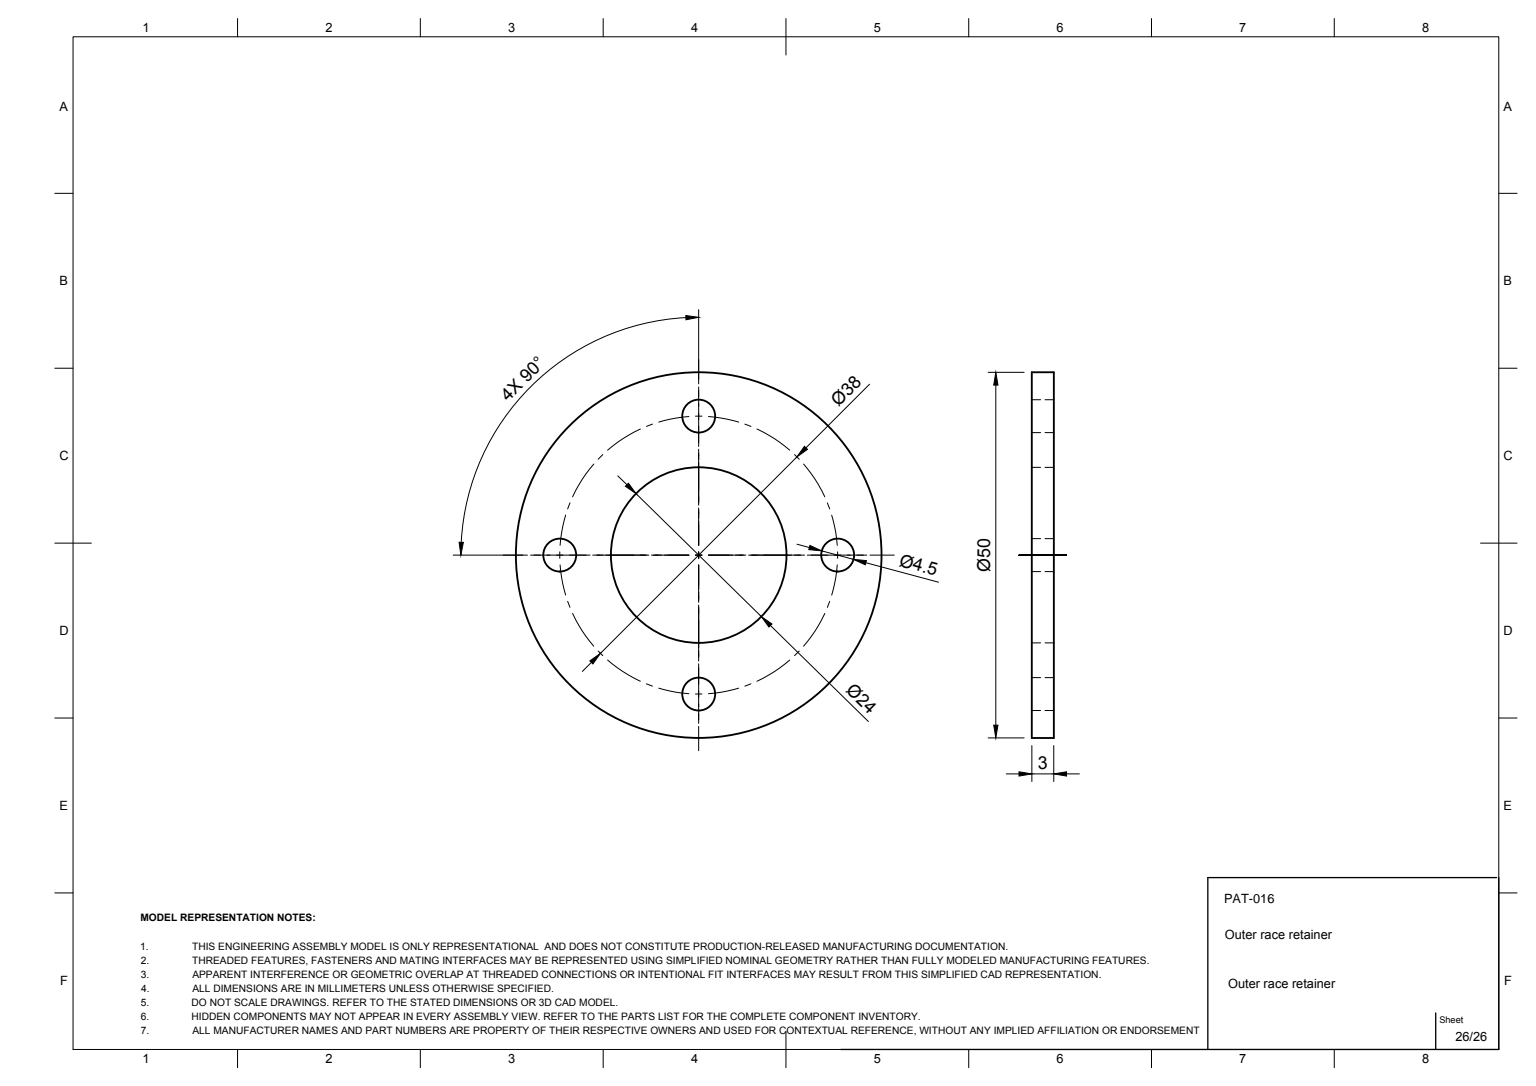
ISO-10303-21;
HEADER;
/* Generated by software containing ST-Developer
 * from STEP Tools, Inc. (www.steptools.com) 
 */

FILE_DESCRIPTION(
/* description */ ('Bracket-mounted idler roller'),
/* implementation_level */ '2;1');

FILE_NAME(
/* name */ 'Outer race retainer.step',
/* time_stamp */ '2026-10-28T03:26:42-07:00',
/* author */ (''),
/* organization */ (''),
/* preprocessor_version */ 'ST-DEVELOPER v20.2',
/* originating_system */ 'Autodesk Translation Framework v15.17.0.0',
/* authorisation */ '');

FILE_SCHEMA (('AUTOMOTIVE_DESIGN { 1 0 10303 214 3 1 1 }'));
ENDSEC;

DATA;
#10=MECHANICAL_DESIGN_GEOMETRIC_PRESENTATION_REPRESENTATION('',(#307),#6241);
#257=SHAPE_REPRESENTATION_RELATIONSHIP('SRR','None',#6363,#278);
#278=ADVANCED_BREP_SHAPE_REPRESENTATION('',(#335),#6239);
#307=STYLED_ITEM('',(#6538),#335);
#335=MANIFOLD_SOLID_BREP('Body1',#3210);
#406=FACE_BOUND('',#950,.T.);
#407=FACE_BOUND('',#951,.T.);
#408=FACE_BOUND('',#952,.T.);
#409=FACE_BOUND('',#953,.T.);
#410=FACE_BOUND('',#954,.T.);
#411=FACE_BOUND('',#956,.T.);
#412=FACE_BOUND('',#957,.T.);
#413=FACE_BOUND('',#958,.T.);
#414=FACE_BOUND('',#959,.T.);
#415=FACE_BOUND('',#960,.T.);
#503=PLANE('',#3819);
#504=PLANE('',#3820);
#682=FACE_OUTER_BOUND('',#943,.T.);
#683=FACE_OUTER_BOUND('',#944,.T.);
#684=FACE_OUTER_BOUND('',#945,.T.);
#685=FACE_OUTER_BOUND('',#946,.T.);
#686=FACE_OUTER_BOUND('',#947,.T.);
#687=FACE_OUTER_BOUND('',#948,.T.);
#688=FACE_OUTER_BOUND('',#949,.T.);
#689=FACE_OUTER_BOUND('',#955,.T.);
#943=EDGE_LOOP('',(#2828,#2829,#2830,#2831));
#944=EDGE_LOOP('',(#2832,#2833,#2834,#2835));
#945=EDGE_LOOP('',(#2836,#2837,#2838,#2839));
#946=EDGE_LOOP('',(#2840,#2841,#2842,#2843));
#947=EDGE_LOOP('',(#2844,#2845,#2846,#2847));
#948=EDGE_LOOP('',(#2848,#2849,#2850,#2851));
#949=EDGE_LOOP('',(#2852));
#950=EDGE_LOOP('',(#2853));
#951=EDGE_LOOP('',(#2854));
#952=EDGE_LOOP('',(#2855));
#953=EDGE_LOOP('',(#2856));
#954=EDGE_LOOP('',(#2857));
#955=EDGE_LOOP('',(#2858));
#956=EDGE_LOOP('',(#2859));
#957=EDGE_LOOP('',(#2860));
#958=EDGE_LOOP('',(#2861));
#959=EDGE_LOOP('',(#2862));
#960=EDGE_LOOP('',(#2863));
#1131=LINE('',#6047,#1313);
#1132=LINE('',#6053,#1314);
#1133=LINE('',#6059,#1315);
#1134=LINE('',#6065,#1316);
#1135=LINE('',#6071,#1317);
#1136=LINE('',#6077,#1318);
#1313=VECTOR('',#4754,0.225);
#1314=VECTOR('',#4761,0.225);
#1315=VECTOR('',#4768,0.225);
#1316=VECTOR('',#4775,0.225);
#1317=VECTOR('',#4782,1.2);
#1318=VECTOR('',#4789,2.5);
#1504=CIRCLE('',#3802,0.225);
#1505=CIRCLE('',#3803,0.225);
#1506=CIRCLE('',#3805,0.225);
#1507=CIRCLE('',#3806,0.225);
#1508=CIRCLE('',#3808,0.225);
#1509=CIRCLE('',#3809,0.225);
#1510=CIRCLE('',#3811,0.225);
#1511=CIRCLE('',#3812,0.225);
#1512=CIRCLE('',#3814,1.2);
#1513=CIRCLE('',#3815,1.2);
#1514=CIRCLE('',#3817,2.5);
#1515=CIRCLE('',#3818,2.5);
#1753=VERTEX_POINT('',#6044);
#1754=VERTEX_POINT('',#6046);
#1755=VERTEX_POINT('',#6050);
#1756=VERTEX_POINT('',#6052);
#1757=VERTEX_POINT('',#6056);
#1758=VERTEX_POINT('',#6058);
#1759=VERTEX_POINT('',#6062);
#1760=VERTEX_POINT('',#6064);
#1761=VERTEX_POINT('',#6068);
#1762=VERTEX_POINT('',#6070);
#1763=VERTEX_POINT('',#6074);
#1764=VERTEX_POINT('',#6076);
#2116=EDGE_CURVE('',#1753,#1753,#1504,.T.);
#2117=EDGE_CURVE('',#1753,#1754,#1131,.T.);
#2118=EDGE_CURVE('',#1754,#1754,#1505,.T.);
#2119=EDGE_CURVE('',#1755,#1755,#1506,.T.);
#2120=EDGE_CURVE('',#1755,#1756,#1132,.T.);
#2121=EDGE_CURVE('',#1756,#1756,#1507,.T.);
#2122=EDGE_CURVE('',#1757,#1757,#1508,.T.);
#2123=EDGE_CURVE('',#1757,#1758,#1133,.T.);
#2124=EDGE_CURVE('',#1758,#1758,#1509,.T.);
#2125=EDGE_CURVE('',#1759,#1759,#1510,.T.);
#2126=EDGE_CURVE('',#1759,#1760,#1134,.T.);
#2127=EDGE_CURVE('',#1760,#1760,#1511,.T.);
#2128=EDGE_CURVE('',#1761,#1761,#1512,.T.);
#2129=EDGE_CURVE('',#1761,#1762,#1135,.T.);
#2130=EDGE_CURVE('',#1762,#1762,#1513,.T.);
#2131=EDGE_CURVE('',#1763,#1763,#1514,.T.);
#2132=EDGE_CURVE('',#1763,#1764,#1136,.T.);
#2133=EDGE_CURVE('',#1764,#1764,#1515,.T.);
#2828=ORIENTED_EDGE('',*,*,#2116,.F.);
#2829=ORIENTED_EDGE('',*,*,#2117,.T.);
#2830=ORIENTED_EDGE('',*,*,#2118,.F.);
#2831=ORIENTED_EDGE('',*,*,#2117,.F.);
#2832=ORIENTED_EDGE('',*,*,#2119,.F.);
#2833=ORIENTED_EDGE('',*,*,#2120,.T.);
#2834=ORIENTED_EDGE('',*,*,#2121,.F.);
#2835=ORIENTED_EDGE('',*,*,#2120,.F.);
#2836=ORIENTED_EDGE('',*,*,#2122,.F.);
#2837=ORIENTED_EDGE('',*,*,#2123,.T.);
#2838=ORIENTED_EDGE('',*,*,#2124,.F.);
#2839=ORIENTED_EDGE('',*,*,#2123,.F.);
#2840=ORIENTED_EDGE('',*,*,#2125,.F.);
#2841=ORIENTED_EDGE('',*,*,#2126,.T.);
#2842=ORIENTED_EDGE('',*,*,#2127,.F.);
#2843=ORIENTED_EDGE('',*,*,#2126,.F.);
#2844=ORIENTED_EDGE('',*,*,#2128,.F.);
#2845=ORIENTED_EDGE('',*,*,#2129,.T.);
#2846=ORIENTED_EDGE('',*,*,#2130,.T.);
#2847=ORIENTED_EDGE('',*,*,#2129,.F.);
#2848=ORIENTED_EDGE('',*,*,#2131,.F.);
#2849=ORIENTED_EDGE('',*,*,#2132,.T.);
#2850=ORIENTED_EDGE('',*,*,#2133,.T.);
#2851=ORIENTED_EDGE('',*,*,#2132,.F.);
#2852=ORIENTED_EDGE('',*,*,#2131,.T.);
#2853=ORIENTED_EDGE('',*,*,#2128,.T.);
#2854=ORIENTED_EDGE('',*,*,#2127,.T.);
#2855=ORIENTED_EDGE('',*,*,#2124,.T.);
#2856=ORIENTED_EDGE('',*,*,#2121,.T.);
#2857=ORIENTED_EDGE('',*,*,#2118,.T.);
#2858=ORIENTED_EDGE('',*,*,#2133,.F.);
#2859=ORIENTED_EDGE('',*,*,#2130,.F.);
#2860=ORIENTED_EDGE('',*,*,#2125,.T.);
#2861=ORIENTED_EDGE('',*,*,#2122,.T.);
#2862=ORIENTED_EDGE('',*,*,#2119,.T.);
#2863=ORIENTED_EDGE('',*,*,#2116,.T.);
#2983=CYLINDRICAL_SURFACE('',#3801,0.225);
#2984=CYLINDRICAL_SURFACE('',#3804,0.225);
#2985=CYLINDRICAL_SURFACE('',#3807,0.225);
#2986=CYLINDRICAL_SURFACE('',#3810,0.225);
#2987=CYLINDRICAL_SURFACE('',#3813,1.2);
#2988=CYLINDRICAL_SURFACE('',#3816,2.5);
#3157=ADVANCED_FACE('',(#682),#2983,.F.);
#3158=ADVANCED_FACE('',(#683),#2984,.F.);
#3159=ADVANCED_FACE('',(#684),#2985,.F.);
#3160=ADVANCED_FACE('',(#685),#2986,.F.);
#3161=ADVANCED_FACE('',(#686),#2987,.F.);
#3162=ADVANCED_FACE('',(#687),#2988,.T.);
#3163=ADVANCED_FACE('',(#688,#406,#407,#408,#409,#410),#503,.T.);
#3164=ADVANCED_FACE('',(#689,#411,#412,#413,#414,#415),#504,.F.);
#3210=CLOSED_SHELL('',(#3157,#3158,#3159,#3160,#3161,#3162,#3163,#3164));
#3800=AXIS2_PLACEMENT_3D('',#6042,#4748,#4749);
#3801=AXIS2_PLACEMENT_3D('',#6043,#4750,#4751);
#3802=AXIS2_PLACEMENT_3D('',#6045,#4752,#4753);
#3803=AXIS2_PLACEMENT_3D('',#6048,#4755,#4756);
#3804=AXIS2_PLACEMENT_3D('',#6049,#4757,#4758);
#3805=AXIS2_PLACEMENT_3D('',#6051,#4759,#4760);
#3806=AXIS2_PLACEMENT_3D('',#6054,#4762,#4763);
#3807=AXIS2_PLACEMENT_3D('',#6055,#4764,#4765);
#3808=AXIS2_PLACEMENT_3D('',#6057,#4766,#4767);
#3809=AXIS2_PLACEMENT_3D('',#6060,#4769,#4770);
#3810=AXIS2_PLACEMENT_3D('',#6061,#4771,#4772);
#3811=AXIS2_PLACEMENT_3D('',#6063,#4773,#4774);
#3812=AXIS2_PLACEMENT_3D('',#6066,#4776,#4777);
#3813=AXIS2_PLACEMENT_3D('',#6067,#4778,#4779);
#3814=AXIS2_PLACEMENT_3D('',#6069,#4780,#4781);
#3815=AXIS2_PLACEMENT_3D('',#6072,#4783,#4784);
#3816=AXIS2_PLACEMENT_3D('',#6073,#4785,#4786);
#3817=AXIS2_PLACEMENT_3D('',#6075,#4787,#4788);
#3818=AXIS2_PLACEMENT_3D('',#6078,#4790,#4791);
#3819=AXIS2_PLACEMENT_3D('',#6079,#4792,#4793);
#3820=AXIS2_PLACEMENT_3D('',#6080,#4794,#4795);
#4748=DIRECTION('axis',(0.,0.,1.));
#4749=DIRECTION('refdir',(1.,0.,0.));
#4750=DIRECTION('center_axis',(0.,1.,0.));
#4751=DIRECTION('ref_axis',(1.,0.,0.));
#4752=DIRECTION('center_axis',(0.,1.,0.));
#4753=DIRECTION('ref_axis',(1.,0.,0.));
#4754=DIRECTION('',(0.,1.,0.));
#4755=DIRECTION('center_axis',(0.,-1.,0.));
#4756=DIRECTION('ref_axis',(1.,0.,0.));
#4757=DIRECTION('center_axis',(0.,1.,0.));
#4758=DIRECTION('ref_axis',(1.,0.,0.));
#4759=DIRECTION('center_axis',(0.,1.,0.));
#4760=DIRECTION('ref_axis',(1.,0.,0.));
#4761=DIRECTION('',(0.,1.,0.));
#4762=DIRECTION('center_axis',(0.,-1.,0.));
#4763=DIRECTION('ref_axis',(1.,0.,0.));
#4764=DIRECTION('center_axis',(0.,1.,0.));
#4765=DIRECTION('ref_axis',(1.,0.,0.));
#4766=DIRECTION('center_axis',(0.,1.,0.));
#4767=DIRECTION('ref_axis',(1.,0.,0.));
#4768=DIRECTION('',(0.,1.,0.));
#4769=DIRECTION('center_axis',(0.,-1.,0.));
#4770=DIRECTION('ref_axis',(1.,0.,0.));
#4771=DIRECTION('center_axis',(0.,1.,0.));
#4772=DIRECTION('ref_axis',(1.,0.,0.));
#4773=DIRECTION('center_axis',(0.,1.,0.));
#4774=DIRECTION('ref_axis',(1.,0.,0.));
#4775=DIRECTION('',(0.,1.,0.));
#4776=DIRECTION('center_axis',(0.,-1.,0.));
#4777=DIRECTION('ref_axis',(1.,0.,0.));
#4778=DIRECTION('center_axis',(0.,1.,0.));
#4779=DIRECTION('ref_axis',(1.,0.,0.));
#4780=DIRECTION('center_axis',(0.,-1.,0.));
#4781=DIRECTION('ref_axis',(1.,0.,0.));
#4782=DIRECTION('',(0.,-1.,0.));
#4783=DIRECTION('center_axis',(0.,-1.,0.));
#4784=DIRECTION('ref_axis',(1.,0.,0.));
#4785=DIRECTION('center_axis',(0.,1.,0.));
#4786=DIRECTION('ref_axis',(1.,0.,0.));
#4787=DIRECTION('center_axis',(0.,1.,0.));
#4788=DIRECTION('ref_axis',(1.,0.,0.));
#4789=DIRECTION('',(0.,-1.,0.));
#4790=DIRECTION('center_axis',(0.,1.,0.));
#4791=DIRECTION('ref_axis',(1.,0.,0.));
#4792=DIRECTION('center_axis',(0.,1.,0.));
#4793=DIRECTION('ref_axis',(1.,0.,0.));
#4794=DIRECTION('center_axis',(0.,1.,0.));
#4795=DIRECTION('ref_axis',(1.,0.,0.));
#6042=CARTESIAN_POINT('',(0.,0.,0.));
#6043=CARTESIAN_POINT('Origin',(-1.9,-0.4,4.5));
#6044=CARTESIAN_POINT('',(-2.125,-0.3,4.5));
#6045=CARTESIAN_POINT('Origin',(-1.9,-0.3,4.5));
#6046=CARTESIAN_POINT('',(-2.125,0.,4.5));
#6047=CARTESIAN_POINT('',(-2.125,-0.4,4.5));
#6048=CARTESIAN_POINT('Origin',(-1.9,0.,4.5));
#6049=CARTESIAN_POINT('Origin',(1.16341445918999E-16,-0.4,6.4));
#6050=CARTESIAN_POINT('',(-0.225,-0.3,6.4));
#6051=CARTESIAN_POINT('Origin',(1.16341445918999E-16,-0.3,6.4));
#6052=CARTESIAN_POINT('',(-0.225,0.,6.4));
#6053=CARTESIAN_POINT('',(-0.225,-0.4,6.4));
#6054=CARTESIAN_POINT('Origin',(1.16341445918999E-16,0.,6.4));
#6055=CARTESIAN_POINT('Origin',(1.9,-0.4,4.5));
#6056=CARTESIAN_POINT('',(1.675,-0.3,4.5));
#6057=CARTESIAN_POINT('Origin',(1.9,-0.3,4.5));
#6058=CARTESIAN_POINT('',(1.675,0.,4.5));
#6059=CARTESIAN_POINT('',(1.675,-0.4,4.5));
#6060=CARTESIAN_POINT('Origin',(1.9,0.,4.5));
#6061=CARTESIAN_POINT('Origin',(-3.49024337756996E-16,-0.4,2.6));
#6062=CARTESIAN_POINT('',(-0.225,-0.3,2.6));
#6063=CARTESIAN_POINT('Origin',(-3.49024337756996E-16,-0.3,2.6));
#6064=CARTESIAN_POINT('',(-0.225,0.,2.6));
#6065=CARTESIAN_POINT('',(-0.225,-0.4,2.6));
#6066=CARTESIAN_POINT('Origin',(-3.49024337756996E-16,0.,2.6));
#6067=CARTESIAN_POINT('Origin',(0.,-0.3,4.5));
#6068=CARTESIAN_POINT('',(-1.2,0.,4.5));
#6069=CARTESIAN_POINT('Origin',(0.,0.,4.5));
#6070=CARTESIAN_POINT('',(-1.2,-0.3,4.5));
#6071=CARTESIAN_POINT('',(-1.2,-0.3,4.5));
#6072=CARTESIAN_POINT('Origin',(0.,-0.3,4.5));
#6073=CARTESIAN_POINT('Origin',(0.,-0.3,4.5));
#6074=CARTESIAN_POINT('',(-2.5,0.,4.5));
#6075=CARTESIAN_POINT('Origin',(0.,0.,4.5));
#6076=CARTESIAN_POINT('',(-2.5,-0.3,4.5));
#6077=CARTESIAN_POINT('',(-2.5,-0.3,4.5));
#6078=CARTESIAN_POINT('Origin',(0.,-0.3,4.5));
#6079=CARTESIAN_POINT('Origin',(0.,0.,4.5));
#6080=CARTESIAN_POINT('Origin',(0.,-0.3,4.5));
#6213=UNCERTAINTY_MEASURE_WITH_UNIT(LENGTH_MEASURE(0.001),#6242,
'DISTANCE_ACCURACY_VALUE',
'Maximum model space distance between geometric entities at asserted c
onnectivities');
#6215=UNCERTAINTY_MEASURE_WITH_UNIT(LENGTH_MEASURE(0.001),#6242,
'DISTANCE_ACCURACY_VALUE',
'Maximum model space distance between geometric entities at asserted c
onnectivities');
#6239=(
GEOMETRIC_REPRESENTATION_CONTEXT(3)
GLOBAL_UNCERTAINTY_ASSIGNED_CONTEXT((#6213))
GLOBAL_UNIT_ASSIGNED_CONTEXT((#6242,#6244,#6245))
REPRESENTATION_CONTEXT('','3D')
);
#6241=(
GEOMETRIC_REPRESENTATION_CONTEXT(3)
GLOBAL_UNCERTAINTY_ASSIGNED_CONTEXT((#6215))
GLOBAL_UNIT_ASSIGNED_CONTEXT((#6242,#6244,#6245))
REPRESENTATION_CONTEXT('','3D')
);
#6242=(
LENGTH_UNIT()
NAMED_UNIT(*)
SI_UNIT(.CENTI.,.METRE.)
);
#6244=(
NAMED_UNIT(*)
PLANE_ANGLE_UNIT()
SI_UNIT($,.RADIAN.)
);
#6245=(
NAMED_UNIT(*)
SI_UNIT($,.STERADIAN.)
SOLID_ANGLE_UNIT()
);
#6269=SHAPE_DEFINITION_REPRESENTATION(#6299,#6363);
#6299=PRODUCT_DEFINITION_SHAPE('',$,#6389);
#6363=SHAPE_REPRESENTATION('',(#3800),#6239);
#6365=PRODUCT_DEFINITION_CONTEXT('part definition',#6442,'design');
#6389=PRODUCT_DEFINITION('Outer race retainer','Outer race retainer',#6414,
#6365);
#6414=PRODUCT_DEFINITION_FORMATION('',$,#6467);
#6442=APPLICATION_CONTEXT(
'Core Data for Automotive Mechanical Design Process');
#6443=PRODUCT_CONTEXT('part definition',#6442,'mechanical');
#6467=PRODUCT('Outer race retainer','Outer race retainer',
'Outer race retainer',(#6443));
#6532=COLOUR_RGB('Grey',0.48,0.52,0.57);
#6533=FILL_AREA_STYLE_COLOUR('',#6532);
#6534=FILL_AREA_STYLE('',(#6533));
#6535=SURFACE_STYLE_FILL_AREA(#6534);
#6536=SURFACE_SIDE_STYLE('',(#6535));
#6537=SURFACE_STYLE_USAGE(.BOTH.,#6536);
#6538=PRESENTATION_STYLE_ASSIGNMENT((#6537));
ENDSEC;
END-ISO-10303-21;
